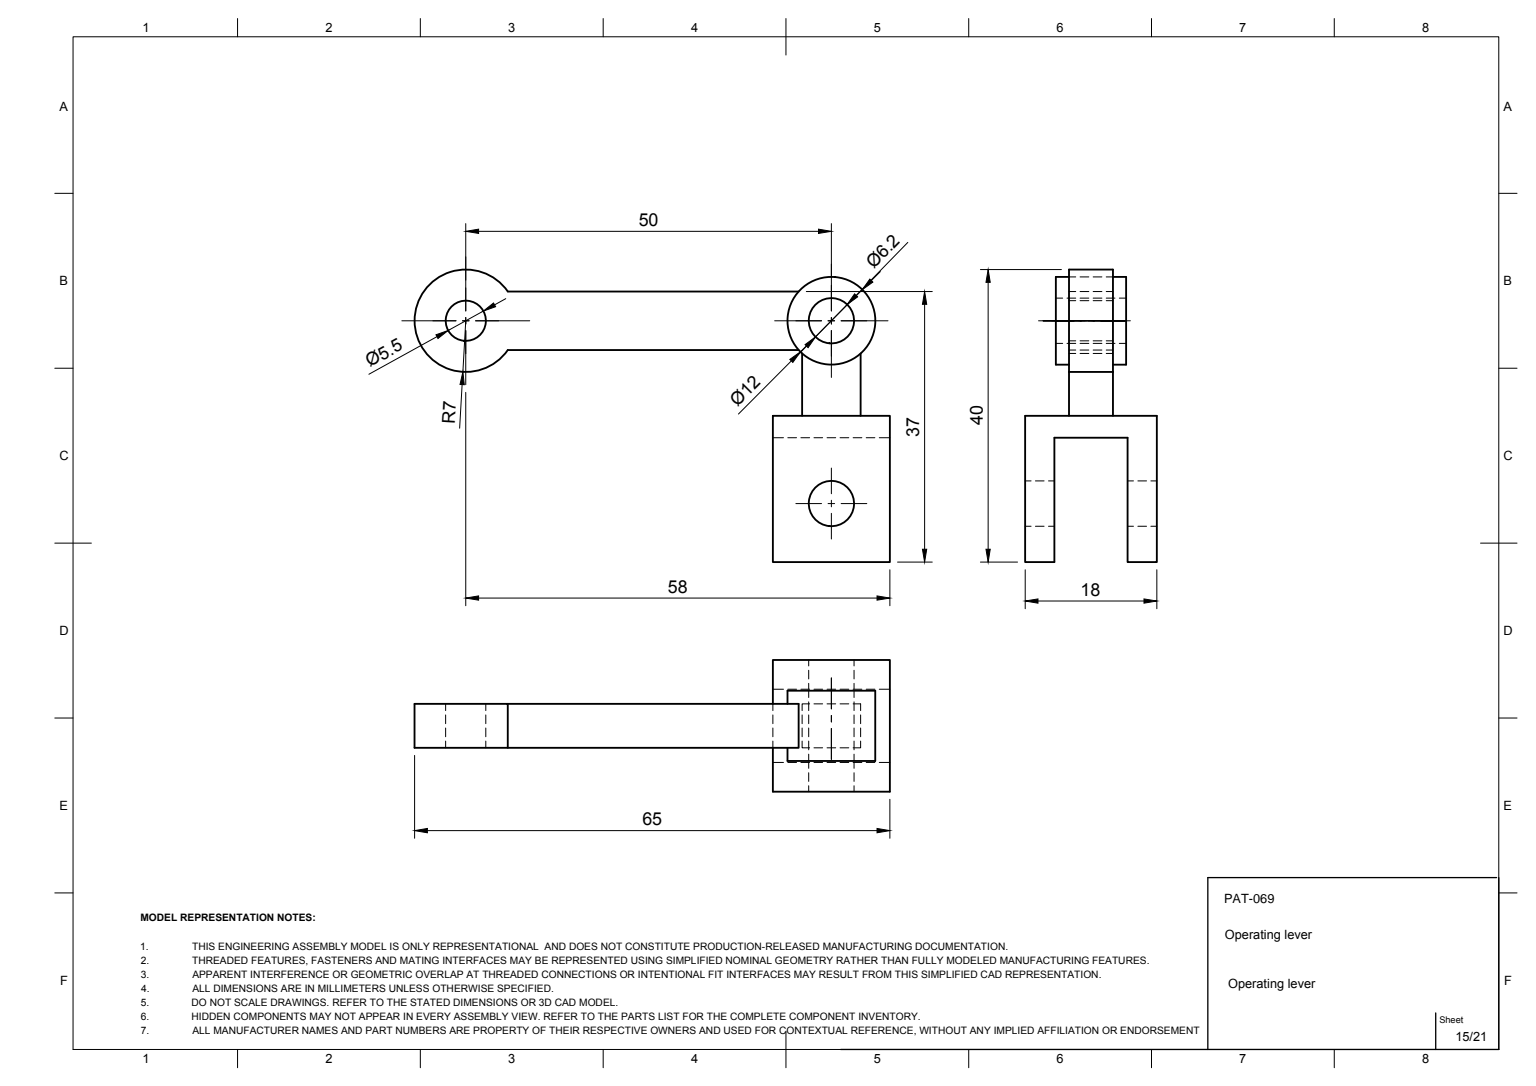
ISO-10303-21;
HEADER;
/* Generated by software containing ST-Developer
 * from STEP Tools, Inc. (www.steptools.com) 
 */

FILE_DESCRIPTION(
/* description */ ('Located fixture plate with toggle clamp'),
/* implementation_level */ '2;1');

FILE_NAME(
/* name */ 'Operating lever.step',
/* time_stamp */ '2026-10-27T21:36:12-07:00',
/* author */ (''),
/* organization */ (''),
/* preprocessor_version */ 'ST-DEVELOPER v20.2',
/* originating_system */ 'Autodesk Translation Framework v15.17.0.0',
/* authorisation */ '');

FILE_SCHEMA (('AUTOMOTIVE_DESIGN { 1 0 10303 214 3 1 1 }'));
ENDSEC;

DATA;
#10=MECHANICAL_DESIGN_GEOMETRIC_PRESENTATION_REPRESENTATION('',(#333),#9285);
#285=SHAPE_REPRESENTATION_RELATIONSHIP('SRR','None',#9409,#309);
#309=ADVANCED_BREP_SHAPE_REPRESENTATION('',(#355),#9271);
#333=STYLED_ITEM('',(#9598),#355);
#355=MANIFOLD_SOLID_BREP('Body1',#5183);
#453=FACE_BOUND('',#1236,.T.);
#454=FACE_BOUND('',#1239,.T.);
#455=FACE_BOUND('',#1245,.T.);
#456=FACE_BOUND('',#1248,.T.);
#457=FACE_BOUND('',#1254,.T.);
#458=FACE_BOUND('',#1255,.T.);
#459=FACE_BOUND('',#1257,.T.);
#460=FACE_BOUND('',#1259,.T.);
#461=FACE_BOUND('',#1262,.T.);
#462=FACE_BOUND('',#1264,.T.);
#463=FACE_BOUND('',#1268,.T.);
#594=PLANE('',#5789);
#595=PLANE('',#5791);
#596=PLANE('',#5792);
#597=PLANE('',#5794);
#598=PLANE('',#5801);
#599=PLANE('',#5802);
#600=PLANE('',#5803);
#601=PLANE('',#5804);
#602=PLANE('',#5805);
#603=PLANE('',#5807);
#604=PLANE('',#5808);
#605=PLANE('',#5810);
#606=PLANE('',#5814);
#607=PLANE('',#5815);
#608=PLANE('',#5816);
#609=PLANE('',#5817);
#610=PLANE('',#5818);
#611=PLANE('',#5819);
#612=PLANE('',#5820);
#613=PLANE('',#5821);
#850=FACE_OUTER_BOUND('',#1232,.T.);
#851=FACE_OUTER_BOUND('',#1233,.T.);
#852=FACE_OUTER_BOUND('',#1234,.T.);
#853=FACE_OUTER_BOUND('',#1235,.T.);
#854=FACE_OUTER_BOUND('',#1237,.T.);
#855=FACE_OUTER_BOUND('',#1238,.T.);
#856=FACE_OUTER_BOUND('',#1240,.T.);
#857=FACE_OUTER_BOUND('',#1241,.T.);
#858=FACE_OUTER_BOUND('',#1242,.T.);
#859=FACE_OUTER_BOUND('',#1243,.T.);
#860=FACE_OUTER_BOUND('',#1244,.T.);
#861=FACE_OUTER_BOUND('',#1246,.T.);
#862=FACE_OUTER_BOUND('',#1247,.T.);
#863=FACE_OUTER_BOUND('',#1249,.T.);
#864=FACE_OUTER_BOUND('',#1250,.T.);
#865=FACE_OUTER_BOUND('',#1251,.T.);
#866=FACE_OUTER_BOUND('',#1252,.T.);
#867=FACE_OUTER_BOUND('',#1253,.T.);
#868=FACE_OUTER_BOUND('',#1256,.T.);
#869=FACE_OUTER_BOUND('',#1258,.T.);
#870=FACE_OUTER_BOUND('',#1260,.T.);
#871=FACE_OUTER_BOUND('',#1261,.T.);
#872=FACE_OUTER_BOUND('',#1263,.T.);
#873=FACE_OUTER_BOUND('',#1265,.T.);
#874=FACE_OUTER_BOUND('',#1266,.T.);
#875=FACE_OUTER_BOUND('',#1267,.T.);
#1232=EDGE_LOOP('',(#4300,#4301,#4302,#4303));
#1233=EDGE_LOOP('',(#4304,#4305,#4306,#4307));
#1234=EDGE_LOOP('',(#4308,#4309,#4310,#4311));
#1235=EDGE_LOOP('',(#4312,#4313,#4314,#4315));
#1236=EDGE_LOOP('',(#4316));
#1237=EDGE_LOOP('',(#4317,#4318,#4319,#4320));
#1238=EDGE_LOOP('',(#4321,#4322,#4323,#4324));
#1239=EDGE_LOOP('',(#4325));
#1240=EDGE_LOOP('',(#4326,#4327,#4328,#4329));
#1241=EDGE_LOOP('',(#4330,#4331,#4332,#4333));
#1242=EDGE_LOOP('',(#4334,#4335,#4336,#4337));
#1243=EDGE_LOOP('',(#4338,#4339,#4340,#4341));
#1244=EDGE_LOOP('',(#4342,#4343,#4344,#4345));
#1245=EDGE_LOOP('',(#4346));
#1246=EDGE_LOOP('',(#4347,#4348,#4349,#4350));
#1247=EDGE_LOOP('',(#4351,#4352,#4353,#4354));
#1248=EDGE_LOOP('',(#4355));
#1249=EDGE_LOOP('',(#4356,#4357,#4358,#4359));
#1250=EDGE_LOOP('',(#4360,#4361,#4362,#4363));
#1251=EDGE_LOOP('',(#4364,#4365,#4366,#4367));
#1252=EDGE_LOOP('',(#4368,#4369,#4370,#4371));
#1253=EDGE_LOOP('',(#4372,#4373,#4374,#4375));
#1254=EDGE_LOOP('',(#4376,#4377,#4378,#4379));
#1255=EDGE_LOOP('',(#4380,#4381,#4382,#4383));
#1256=EDGE_LOOP('',(#4384));
#1257=EDGE_LOOP('',(#4385));
#1258=EDGE_LOOP('',(#4386));
#1259=EDGE_LOOP('',(#4387));
#1260=EDGE_LOOP('',(#4388,#4389,#4390,#4391,#4392,#4393,#4394,#4395));
#1261=EDGE_LOOP('',(#4396,#4397,#4398,#4399));
#1262=EDGE_LOOP('',(#4400));
#1263=EDGE_LOOP('',(#4401,#4402,#4403,#4404));
#1264=EDGE_LOOP('',(#4405,#4406,#4407,#4408));
#1265=EDGE_LOOP('',(#4409,#4410,#4411,#4412));
#1266=EDGE_LOOP('',(#4413,#4414,#4415,#4416,#4417,#4418,#4419,#4420));
#1267=EDGE_LOOP('',(#4421,#4422,#4423,#4424));
#1268=EDGE_LOOP('',(#4425));
#1509=CIRCLE('',#5781,0.275);
#1510=CIRCLE('',#5782,0.275);
#1511=CIRCLE('',#5784,0.31);
#1512=CIRCLE('',#5785,0.31);
#1513=CIRCLE('',#5787,0.7);
#1514=CIRCLE('',#5788,0.7);
#1515=CIRCLE('',#5790,0.6);
#1516=CIRCLE('',#5793,0.6);
#1517=CIRCLE('',#5796,0.31);
#1518=CIRCLE('',#5797,0.31);
#1519=CIRCLE('',#5799,0.31);
#1520=CIRCLE('',#5800,0.31);
#1521=CIRCLE('',#5806,0.6);
#1522=CIRCLE('',#5809,0.6);
#1523=CIRCLE('',#5812,0.6);
#1524=CIRCLE('',#5813,0.6);
#1841=LINE('',#8492,#2251);
#1842=LINE('',#8498,#2252);
#1843=LINE('',#8503,#2253);
#1844=LINE('',#8507,#2254);
#1845=LINE('',#8511,#2255);
#1846=LINE('',#8514,#2256);
#1847=LINE('',#8517,#2257);
#1848=LINE('',#8518,#2258);
#1849=LINE('',#8521,#2259);
#1850=LINE('',#8524,#2260);
#1851=LINE('',#8529,#2261);
#1852=LINE('',#8535,#2262);
#1853=LINE('',#8540,#2263);
#1854=LINE('',#8542,#2264);
#1855=LINE('',#8544,#2265);
#1856=LINE('',#8545,#2266);
#1857=LINE('',#8549,#2267);
#1858=LINE('',#8551,#2268);
#1859=LINE('',#8553,#2269);
#1860=LINE('',#8554,#2270);
#1861=LINE('',#8558,#2271);
#1862=LINE('',#8559,#2272);
#1863=LINE('',#8560,#2273);
#1864=LINE('',#8562,#2274);
#1865=LINE('',#8563,#2275);
#1866=LINE('',#8567,#2276);
#1867=LINE('',#8569,#2277);
#1868=LINE('',#8572,#2278);
#1869=LINE('',#8575,#2279);
#1870=LINE('',#8577,#2280);
#1871=LINE('',#8578,#2281);
#1872=LINE('',#8581,#2282);
#1873=LINE('',#8583,#2283);
#1874=LINE('',#8586,#2284);
#1875=LINE('',#8587,#2285);
#1876=LINE('',#8592,#2286);
#1877=LINE('',#8598,#2287);
#1878=LINE('',#8600,#2288);
#1879=LINE('',#8602,#2289);
#1880=LINE('',#8603,#2290);
#1881=LINE('',#8606,#2291);
#1882=LINE('',#8607,#2292);
#1883=LINE('',#8610,#2293);
#1884=LINE('',#8611,#2294);
#1885=LINE('',#8614,#2295);
#1886=LINE('',#8615,#2296);
#1887=LINE('',#8617,#2297);
#2251=VECTOR('',#6931,0.275);
#2252=VECTOR('',#6938,0.31);
#2253=VECTOR('',#6943,1.);
#2254=VECTOR('',#6946,1.);
#2255=VECTOR('',#6951,1.);
#2256=VECTOR('',#6954,1.);
#2257=VECTOR('',#6957,1.);
#2258=VECTOR('',#6958,1.);
#2259=VECTOR('',#6961,1.);
#2260=VECTOR('',#6966,1.);
#2261=VECTOR('',#6971,0.31);
#2262=VECTOR('',#6978,0.31);
#2263=VECTOR('',#6983,1.);
#2264=VECTOR('',#6984,1.);
#2265=VECTOR('',#6985,1.);
#2266=VECTOR('',#6986,1.);
#2267=VECTOR('',#6989,1.);
#2268=VECTOR('',#6990,1.);
#2269=VECTOR('',#6991,1.);
#2270=VECTOR('',#6992,1.);
#2271=VECTOR('',#6995,1.);
#2272=VECTOR('',#6996,1.);
#2273=VECTOR('',#6997,1.);
#2274=VECTOR('',#7000,1.);
#2275=VECTOR('',#7001,1.);
#2276=VECTOR('',#7004,1.);
#2277=VECTOR('',#7005,1.);
#2278=VECTOR('',#7008,1.);
#2279=VECTOR('',#7011,1.);
#2280=VECTOR('',#7012,1.);
#2281=VECTOR('',#7013,1.);
#2282=VECTOR('',#7016,1.);
#2283=VECTOR('',#7017,1.);
#2284=VECTOR('',#7022,1.);
#2285=VECTOR('',#7023,1.);
#2286=VECTOR('',#7028,0.6);
#2287=VECTOR('',#7037,1.);
#2288=VECTOR('',#7038,1.);
#2289=VECTOR('',#7039,1.);
#2290=VECTOR('',#7040,1.);
#2291=VECTOR('',#7043,1.);
#2292=VECTOR('',#7044,1.);
#2293=VECTOR('',#7047,1.);
#2294=VECTOR('',#7048,1.);
#2295=VECTOR('',#7051,1.);
#2296=VECTOR('',#7052,1.);
#2297=VECTOR('',#7055,1.);
#2669=VERTEX_POINT('',#8489);
#2670=VERTEX_POINT('',#8491);
#2671=VERTEX_POINT('',#8495);
#2672=VERTEX_POINT('',#8497);
#2673=VERTEX_POINT('',#8501);
#2674=VERTEX_POINT('',#8502);
#2675=VERTEX_POINT('',#8504);
#2676=VERTEX_POINT('',#8506);
#2677=VERTEX_POINT('',#8510);
#2678=VERTEX_POINT('',#8512);
#2679=VERTEX_POINT('',#8516);
#2680=VERTEX_POINT('',#8520);
#2681=VERTEX_POINT('',#8526);
#2682=VERTEX_POINT('',#8528);
#2683=VERTEX_POINT('',#8532);
#2684=VERTEX_POINT('',#8534);
#2685=VERTEX_POINT('',#8538);
#2686=VERTEX_POINT('',#8539);
#2687=VERTEX_POINT('',#8541);
#2688=VERTEX_POINT('',#8543);
#2689=VERTEX_POINT('',#8547);
#2690=VERTEX_POINT('',#8548);
#2691=VERTEX_POINT('',#8550);
#2692=VERTEX_POINT('',#8552);
#2693=VERTEX_POINT('',#8556);
#2694=VERTEX_POINT('',#8557);
#2695=VERTEX_POINT('',#8565);
#2696=VERTEX_POINT('',#8566);
#2697=VERTEX_POINT('',#8568);
#2698=VERTEX_POINT('',#8570);
#2699=VERTEX_POINT('',#8574);
#2700=VERTEX_POINT('',#8576);
#2701=VERTEX_POINT('',#8580);
#2702=VERTEX_POINT('',#8582);
#2703=VERTEX_POINT('',#8589);
#2704=VERTEX_POINT('',#8591);
#2705=VERTEX_POINT('',#8597);
#2706=VERTEX_POINT('',#8599);
#2707=VERTEX_POINT('',#8601);
#2708=VERTEX_POINT('',#8605);
#2709=VERTEX_POINT('',#8609);
#2710=VERTEX_POINT('',#8613);
#3238=EDGE_CURVE('',#2669,#2669,#1509,.T.);
#3239=EDGE_CURVE('',#2669,#2670,#1841,.T.);
#3240=EDGE_CURVE('',#2670,#2670,#1510,.T.);
#3241=EDGE_CURVE('',#2671,#2671,#1511,.T.);
#3242=EDGE_CURVE('',#2671,#2672,#1842,.T.);
#3243=EDGE_CURVE('',#2672,#2672,#1512,.T.);
#3244=EDGE_CURVE('',#2673,#2674,#1843,.T.);
#3245=EDGE_CURVE('',#2675,#2673,#1513,.T.);
#3246=EDGE_CURVE('',#2676,#2675,#1844,.T.);
#3247=EDGE_CURVE('',#2676,#2674,#1514,.T.);
#3248=EDGE_CURVE('',#2677,#2676,#1845,.T.);
#3249=EDGE_CURVE('',#2678,#2677,#1515,.T.);
#3250=EDGE_CURVE('',#2674,#2678,#1846,.T.);
#3251=EDGE_CURVE('',#2679,#2675,#1847,.T.);
#3252=EDGE_CURVE('',#2677,#2679,#1848,.T.);
#3253=EDGE_CURVE('',#2673,#2680,#1849,.T.);
#3254=EDGE_CURVE('',#2679,#2680,#1516,.T.);
#3255=EDGE_CURVE('',#2680,#2678,#1850,.T.);
#3256=EDGE_CURVE('',#2681,#2681,#1517,.T.);
#3257=EDGE_CURVE('',#2681,#2682,#1851,.T.);
#3258=EDGE_CURVE('',#2682,#2682,#1518,.T.);
#3259=EDGE_CURVE('',#2683,#2683,#1519,.T.);
#3260=EDGE_CURVE('',#2683,#2684,#1852,.T.);
#3261=EDGE_CURVE('',#2684,#2684,#1520,.T.);
#3262=EDGE_CURVE('',#2685,#2686,#1853,.T.);
#3263=EDGE_CURVE('',#2685,#2687,#1854,.T.);
#3264=EDGE_CURVE('',#2688,#2687,#1855,.T.);
#3265=EDGE_CURVE('',#2686,#2688,#1856,.T.);
#3266=EDGE_CURVE('',#2689,#2690,#1857,.T.);
#3267=EDGE_CURVE('',#2690,#2691,#1858,.T.);
#3268=EDGE_CURVE('',#2691,#2692,#1859,.T.);
#3269=EDGE_CURVE('',#2692,#2689,#1860,.T.);
#3270=EDGE_CURVE('',#2693,#2694,#1861,.T.);
#3271=EDGE_CURVE('',#2693,#2691,#1862,.T.);
#3272=EDGE_CURVE('',#2694,#2690,#1863,.T.);
#3273=EDGE_CURVE('',#2687,#2693,#1864,.T.);
#3274=EDGE_CURVE('',#2694,#2688,#1865,.T.);
#3275=EDGE_CURVE('',#2695,#2696,#1866,.T.);
#3276=EDGE_CURVE('',#2697,#2696,#1867,.T.);
#3277=EDGE_CURVE('',#2698,#2697,#1521,.T.);
#3278=EDGE_CURVE('',#2695,#2698,#1868,.T.);
#3279=EDGE_CURVE('',#2696,#2699,#1869,.T.);
#3280=EDGE_CURVE('',#2700,#2699,#1870,.T.);
#3281=EDGE_CURVE('',#2697,#2700,#1871,.T.);
#3282=EDGE_CURVE('',#2699,#2701,#1872,.T.);
#3283=EDGE_CURVE('',#2701,#2702,#1873,.T.);
#3284=EDGE_CURVE('',#2700,#2702,#1522,.T.);
#3285=EDGE_CURVE('',#2701,#2695,#1874,.T.);
#3286=EDGE_CURVE('',#2702,#2698,#1875,.T.);
#3287=EDGE_CURVE('',#2703,#2703,#1523,.T.);
#3288=EDGE_CURVE('',#2703,#2704,#1876,.T.);
#3289=EDGE_CURVE('',#2704,#2704,#1524,.T.);
#3290=EDGE_CURVE('',#2705,#2685,#1877,.T.);
#3291=EDGE_CURVE('',#2706,#2705,#1878,.T.);
#3292=EDGE_CURVE('',#2707,#2706,#1879,.T.);
#3293=EDGE_CURVE('',#2707,#2692,#1880,.T.);
#3294=EDGE_CURVE('',#2686,#2708,#1881,.T.);
#3295=EDGE_CURVE('',#2708,#2705,#1882,.T.);
#3296=EDGE_CURVE('',#2709,#2707,#1883,.T.);
#3297=EDGE_CURVE('',#2709,#2689,#1884,.T.);
#3298=EDGE_CURVE('',#2706,#2710,#1885,.T.);
#3299=EDGE_CURVE('',#2710,#2708,#1886,.T.);
#3300=EDGE_CURVE('',#2710,#2709,#1887,.T.);
#4300=ORIENTED_EDGE('',*,*,#3238,.F.);
#4301=ORIENTED_EDGE('',*,*,#3239,.T.);
#4302=ORIENTED_EDGE('',*,*,#3240,.F.);
#4303=ORIENTED_EDGE('',*,*,#3239,.F.);
#4304=ORIENTED_EDGE('',*,*,#3241,.F.);
#4305=ORIENTED_EDGE('',*,*,#3242,.T.);
#4306=ORIENTED_EDGE('',*,*,#3243,.F.);
#4307=ORIENTED_EDGE('',*,*,#3242,.F.);
#4308=ORIENTED_EDGE('',*,*,#3244,.F.);
#4309=ORIENTED_EDGE('',*,*,#3245,.F.);
#4310=ORIENTED_EDGE('',*,*,#3246,.F.);
#4311=ORIENTED_EDGE('',*,*,#3247,.T.);
#4312=ORIENTED_EDGE('',*,*,#3247,.F.);
#4313=ORIENTED_EDGE('',*,*,#3248,.F.);
#4314=ORIENTED_EDGE('',*,*,#3249,.F.);
#4315=ORIENTED_EDGE('',*,*,#3250,.F.);
#4316=ORIENTED_EDGE('',*,*,#3238,.T.);
#4317=ORIENTED_EDGE('',*,*,#3246,.T.);
#4318=ORIENTED_EDGE('',*,*,#3251,.F.);
#4319=ORIENTED_EDGE('',*,*,#3252,.F.);
#4320=ORIENTED_EDGE('',*,*,#3248,.T.);
#4321=ORIENTED_EDGE('',*,*,#3253,.T.);
#4322=ORIENTED_EDGE('',*,*,#3254,.F.);
#4323=ORIENTED_EDGE('',*,*,#3251,.T.);
#4324=ORIENTED_EDGE('',*,*,#3245,.T.);
#4325=ORIENTED_EDGE('',*,*,#3240,.T.);
#4326=ORIENTED_EDGE('',*,*,#3244,.T.);
#4327=ORIENTED_EDGE('',*,*,#3250,.T.);
#4328=ORIENTED_EDGE('',*,*,#3255,.F.);
#4329=ORIENTED_EDGE('',*,*,#3253,.F.);
#4330=ORIENTED_EDGE('',*,*,#3256,.F.);
#4331=ORIENTED_EDGE('',*,*,#3257,.T.);
#4332=ORIENTED_EDGE('',*,*,#3258,.F.);
#4333=ORIENTED_EDGE('',*,*,#3257,.F.);
#4334=ORIENTED_EDGE('',*,*,#3259,.F.);
#4335=ORIENTED_EDGE('',*,*,#3260,.T.);
#4336=ORIENTED_EDGE('',*,*,#3261,.F.);
#4337=ORIENTED_EDGE('',*,*,#3260,.F.);
#4338=ORIENTED_EDGE('',*,*,#3262,.F.);
#4339=ORIENTED_EDGE('',*,*,#3263,.T.);
#4340=ORIENTED_EDGE('',*,*,#3264,.F.);
#4341=ORIENTED_EDGE('',*,*,#3265,.F.);
#4342=ORIENTED_EDGE('',*,*,#3266,.T.);
#4343=ORIENTED_EDGE('',*,*,#3267,.T.);
#4344=ORIENTED_EDGE('',*,*,#3268,.T.);
#4345=ORIENTED_EDGE('',*,*,#3269,.T.);
#4346=ORIENTED_EDGE('',*,*,#3261,.T.);
#4347=ORIENTED_EDGE('',*,*,#3270,.F.);
#4348=ORIENTED_EDGE('',*,*,#3271,.T.);
#4349=ORIENTED_EDGE('',*,*,#3267,.F.);
#4350=ORIENTED_EDGE('',*,*,#3272,.F.);
#4351=ORIENTED_EDGE('',*,*,#3264,.T.);
#4352=ORIENTED_EDGE('',*,*,#3273,.T.);
#4353=ORIENTED_EDGE('',*,*,#3270,.T.);
#4354=ORIENTED_EDGE('',*,*,#3274,.T.);
#4355=ORIENTED_EDGE('',*,*,#3259,.T.);
#4356=ORIENTED_EDGE('',*,*,#3275,.T.);
#4357=ORIENTED_EDGE('',*,*,#3276,.F.);
#4358=ORIENTED_EDGE('',*,*,#3277,.F.);
#4359=ORIENTED_EDGE('',*,*,#3278,.F.);
#4360=ORIENTED_EDGE('',*,*,#3279,.T.);
#4361=ORIENTED_EDGE('',*,*,#3280,.F.);
#4362=ORIENTED_EDGE('',*,*,#3281,.F.);
#4363=ORIENTED_EDGE('',*,*,#3276,.T.);
#4364=ORIENTED_EDGE('',*,*,#3282,.T.);
#4365=ORIENTED_EDGE('',*,*,#3283,.T.);
#4366=ORIENTED_EDGE('',*,*,#3284,.F.);
#4367=ORIENTED_EDGE('',*,*,#3280,.T.);
#4368=ORIENTED_EDGE('',*,*,#3285,.T.);
#4369=ORIENTED_EDGE('',*,*,#3278,.T.);
#4370=ORIENTED_EDGE('',*,*,#3286,.F.);
#4371=ORIENTED_EDGE('',*,*,#3283,.F.);
#4372=ORIENTED_EDGE('',*,*,#3287,.F.);
#4373=ORIENTED_EDGE('',*,*,#3288,.T.);
#4374=ORIENTED_EDGE('',*,*,#3289,.T.);
#4375=ORIENTED_EDGE('',*,*,#3288,.F.);
#4376=ORIENTED_EDGE('',*,*,#3252,.T.);
#4377=ORIENTED_EDGE('',*,*,#3254,.T.);
#4378=ORIENTED_EDGE('',*,*,#3255,.T.);
#4379=ORIENTED_EDGE('',*,*,#3249,.T.);
#4380=ORIENTED_EDGE('',*,*,#3281,.T.);
#4381=ORIENTED_EDGE('',*,*,#3284,.T.);
#4382=ORIENTED_EDGE('',*,*,#3286,.T.);
#4383=ORIENTED_EDGE('',*,*,#3277,.T.);
#4384=ORIENTED_EDGE('',*,*,#3287,.T.);
#4385=ORIENTED_EDGE('',*,*,#3243,.T.);
#4386=ORIENTED_EDGE('',*,*,#3289,.F.);
#4387=ORIENTED_EDGE('',*,*,#3241,.T.);
#4388=ORIENTED_EDGE('',*,*,#3290,.F.);
#4389=ORIENTED_EDGE('',*,*,#3291,.F.);
#4390=ORIENTED_EDGE('',*,*,#3292,.F.);
#4391=ORIENTED_EDGE('',*,*,#3293,.T.);
#4392=ORIENTED_EDGE('',*,*,#3268,.F.);
#4393=ORIENTED_EDGE('',*,*,#3271,.F.);
#4394=ORIENTED_EDGE('',*,*,#3273,.F.);
#4395=ORIENTED_EDGE('',*,*,#3263,.F.);
#4396=ORIENTED_EDGE('',*,*,#3262,.T.);
#4397=ORIENTED_EDGE('',*,*,#3294,.T.);
#4398=ORIENTED_EDGE('',*,*,#3295,.T.);
#4399=ORIENTED_EDGE('',*,*,#3290,.T.);
#4400=ORIENTED_EDGE('',*,*,#3258,.T.);
#4401=ORIENTED_EDGE('',*,*,#3296,.F.);
#4402=ORIENTED_EDGE('',*,*,#3297,.T.);
#4403=ORIENTED_EDGE('',*,*,#3269,.F.);
#4404=ORIENTED_EDGE('',*,*,#3293,.F.);
#4405=ORIENTED_EDGE('',*,*,#3282,.F.);
#4406=ORIENTED_EDGE('',*,*,#3279,.F.);
#4407=ORIENTED_EDGE('',*,*,#3275,.F.);
#4408=ORIENTED_EDGE('',*,*,#3285,.F.);
#4409=ORIENTED_EDGE('',*,*,#3298,.F.);
#4410=ORIENTED_EDGE('',*,*,#3291,.T.);
#4411=ORIENTED_EDGE('',*,*,#3295,.F.);
#4412=ORIENTED_EDGE('',*,*,#3299,.F.);
#4413=ORIENTED_EDGE('',*,*,#3300,.F.);
#4414=ORIENTED_EDGE('',*,*,#3299,.T.);
#4415=ORIENTED_EDGE('',*,*,#3294,.F.);
#4416=ORIENTED_EDGE('',*,*,#3265,.T.);
#4417=ORIENTED_EDGE('',*,*,#3274,.F.);
#4418=ORIENTED_EDGE('',*,*,#3272,.T.);
#4419=ORIENTED_EDGE('',*,*,#3266,.F.);
#4420=ORIENTED_EDGE('',*,*,#3297,.F.);
#4421=ORIENTED_EDGE('',*,*,#3292,.T.);
#4422=ORIENTED_EDGE('',*,*,#3298,.T.);
#4423=ORIENTED_EDGE('',*,*,#3300,.T.);
#4424=ORIENTED_EDGE('',*,*,#3296,.T.);
#4425=ORIENTED_EDGE('',*,*,#3256,.T.);
#4845=CYLINDRICAL_SURFACE('',#5780,0.275);
#4846=CYLINDRICAL_SURFACE('',#5783,0.31);
#4847=CYLINDRICAL_SURFACE('',#5786,0.7);
#4848=CYLINDRICAL_SURFACE('',#5795,0.31);
#4849=CYLINDRICAL_SURFACE('',#5798,0.31);
#4850=CYLINDRICAL_SURFACE('',#5811,0.6);
#5051=ADVANCED_FACE('',(#850),#4845,.F.);
#5052=ADVANCED_FACE('',(#851),#4846,.F.);
#5053=ADVANCED_FACE('',(#852),#4847,.T.);
#5054=ADVANCED_FACE('',(#853,#453),#594,.F.);
#5055=ADVANCED_FACE('',(#854),#595,.T.);
#5056=ADVANCED_FACE('',(#855,#454),#596,.T.);
#5057=ADVANCED_FACE('',(#856),#597,.T.);
#5058=ADVANCED_FACE('',(#857),#4848,.F.);
#5059=ADVANCED_FACE('',(#858),#4849,.F.);
#5060=ADVANCED_FACE('',(#859),#598,.T.);
#5061=ADVANCED_FACE('',(#860,#455),#599,.T.);
#5062=ADVANCED_FACE('',(#861),#600,.T.);
#5063=ADVANCED_FACE('',(#862,#456),#601,.F.);
#5064=ADVANCED_FACE('',(#863),#602,.F.);
#5065=ADVANCED_FACE('',(#864),#603,.T.);
#5066=ADVANCED_FACE('',(#865),#604,.T.);
#5067=ADVANCED_FACE('',(#866),#605,.T.);
#5068=ADVANCED_FACE('',(#867,#457,#458),#4850,.T.);
#5069=ADVANCED_FACE('',(#868,#459),#606,.T.);
#5070=ADVANCED_FACE('',(#869,#460),#607,.F.);
#5071=ADVANCED_FACE('',(#870),#608,.T.);
#5072=ADVANCED_FACE('',(#871,#461),#609,.T.);
#5073=ADVANCED_FACE('',(#872,#462),#610,.T.);
#5074=ADVANCED_FACE('',(#873),#611,.T.);
#5075=ADVANCED_FACE('',(#874),#612,.T.);
#5076=ADVANCED_FACE('',(#875,#463),#613,.F.);
#5183=CLOSED_SHELL('',(#5051,#5052,#5053,#5054,#5055,#5056,#5057,#5058,
#5059,#5060,#5061,#5062,#5063,#5064,#5065,#5066,#5067,#5068,#5069,#5070,
#5071,#5072,#5073,#5074,#5075,#5076));
#5779=AXIS2_PLACEMENT_3D('',#8487,#6925,#6926);
#5780=AXIS2_PLACEMENT_3D('',#8488,#6927,#6928);
#5781=AXIS2_PLACEMENT_3D('',#8490,#6929,#6930);
#5782=AXIS2_PLACEMENT_3D('',#8493,#6932,#6933);
#5783=AXIS2_PLACEMENT_3D('',#8494,#6934,#6935);
#5784=AXIS2_PLACEMENT_3D('',#8496,#6936,#6937);
#5785=AXIS2_PLACEMENT_3D('',#8499,#6939,#6940);
#5786=AXIS2_PLACEMENT_3D('',#8500,#6941,#6942);
#5787=AXIS2_PLACEMENT_3D('',#8505,#6944,#6945);
#5788=AXIS2_PLACEMENT_3D('',#8508,#6947,#6948);
#5789=AXIS2_PLACEMENT_3D('',#8509,#6949,#6950);
#5790=AXIS2_PLACEMENT_3D('',#8513,#6952,#6953);
#5791=AXIS2_PLACEMENT_3D('',#8515,#6955,#6956);
#5792=AXIS2_PLACEMENT_3D('',#8519,#6959,#6960);
#5793=AXIS2_PLACEMENT_3D('',#8522,#6962,#6963);
#5794=AXIS2_PLACEMENT_3D('',#8523,#6964,#6965);
#5795=AXIS2_PLACEMENT_3D('',#8525,#6967,#6968);
#5796=AXIS2_PLACEMENT_3D('',#8527,#6969,#6970);
#5797=AXIS2_PLACEMENT_3D('',#8530,#6972,#6973);
#5798=AXIS2_PLACEMENT_3D('',#8531,#6974,#6975);
#5799=AXIS2_PLACEMENT_3D('',#8533,#6976,#6977);
#5800=AXIS2_PLACEMENT_3D('',#8536,#6979,#6980);
#5801=AXIS2_PLACEMENT_3D('',#8537,#6981,#6982);
#5802=AXIS2_PLACEMENT_3D('',#8546,#6987,#6988);
#5803=AXIS2_PLACEMENT_3D('',#8555,#6993,#6994);
#5804=AXIS2_PLACEMENT_3D('',#8561,#6998,#6999);
#5805=AXIS2_PLACEMENT_3D('',#8564,#7002,#7003);
#5806=AXIS2_PLACEMENT_3D('',#8571,#7006,#7007);
#5807=AXIS2_PLACEMENT_3D('',#8573,#7009,#7010);
#5808=AXIS2_PLACEMENT_3D('',#8579,#7014,#7015);
#5809=AXIS2_PLACEMENT_3D('',#8584,#7018,#7019);
#5810=AXIS2_PLACEMENT_3D('',#8585,#7020,#7021);
#5811=AXIS2_PLACEMENT_3D('',#8588,#7024,#7025);
#5812=AXIS2_PLACEMENT_3D('',#8590,#7026,#7027);
#5813=AXIS2_PLACEMENT_3D('',#8593,#7029,#7030);
#5814=AXIS2_PLACEMENT_3D('',#8594,#7031,#7032);
#5815=AXIS2_PLACEMENT_3D('',#8595,#7033,#7034);
#5816=AXIS2_PLACEMENT_3D('',#8596,#7035,#7036);
#5817=AXIS2_PLACEMENT_3D('',#8604,#7041,#7042);
#5818=AXIS2_PLACEMENT_3D('',#8608,#7045,#7046);
#5819=AXIS2_PLACEMENT_3D('',#8612,#7049,#7050);
#5820=AXIS2_PLACEMENT_3D('',#8616,#7053,#7054);
#5821=AXIS2_PLACEMENT_3D('',#8618,#7056,#7057);
#6925=DIRECTION('axis',(0.,0.,1.));
#6926=DIRECTION('refdir',(1.,0.,0.));
#6927=DIRECTION('center_axis',(0.,1.,0.));
#6928=DIRECTION('ref_axis',(1.,0.,0.));
#6929=DIRECTION('center_axis',(0.,1.,0.));
#6930=DIRECTION('ref_axis',(1.,0.,0.));
#6931=DIRECTION('',(0.,1.,0.));
#6932=DIRECTION('center_axis',(0.,-1.,0.));
#6933=DIRECTION('ref_axis',(1.,0.,0.));
#6934=DIRECTION('center_axis',(0.,1.,0.));
#6935=DIRECTION('ref_axis',(1.,0.,0.));
#6936=DIRECTION('center_axis',(0.,1.,0.));
#6937=DIRECTION('ref_axis',(1.,0.,0.));
#6938=DIRECTION('',(0.,1.,0.));
#6939=DIRECTION('center_axis',(0.,-1.,0.));
#6940=DIRECTION('ref_axis',(1.,0.,0.));
#6941=DIRECTION('center_axis',(0.,1.,0.));
#6942=DIRECTION('ref_axis',(0.0871557427476581,0.,0.996194698091746));
#6943=DIRECTION('',(0.,-1.,0.));
#6944=DIRECTION('center_axis',(0.,1.,0.));
#6945=DIRECTION('ref_axis',(1.,0.,0.));
#6946=DIRECTION('',(0.,1.,0.));
#6947=DIRECTION('center_axis',(0.,1.,0.));
#6948=DIRECTION('ref_axis',(1.,0.,0.));
#6949=DIRECTION('center_axis',(0.,1.,0.));
#6950=DIRECTION('ref_axis',(1.,0.,0.));
#6951=DIRECTION('',(0.0871557427476582,0.,0.996194698091746));
#6952=DIRECTION('center_axis',(0.,-1.,0.));
#6953=DIRECTION('ref_axis',(1.,0.,0.));
#6954=DIRECTION('',(-0.0871557427476581,0.,-0.996194698091746));
#6955=DIRECTION('center_axis',(-0.996194698091746,0.,0.0871557427476582));
#6956=DIRECTION('ref_axis',(0.0871557427476582,0.,0.996194698091746));
#6957=DIRECTION('',(0.0871557427476582,0.,0.996194698091746));
#6958=DIRECTION('',(0.,1.,0.));
#6959=DIRECTION('center_axis',(0.,1.,0.));
#6960=DIRECTION('ref_axis',(0.,0.,1.));
#6961=DIRECTION('',(-0.0871557427476581,0.,-0.996194698091746));
#6962=DIRECTION('center_axis',(0.,1.,0.));
#6963=DIRECTION('ref_axis',(1.,0.,0.));
#6964=DIRECTION('center_axis',(0.996194698091746,0.,-0.0871557427476581));
#6965=DIRECTION('ref_axis',(-0.0871557427476581,0.,-0.996194698091746));
#6966=DIRECTION('',(0.,-1.,0.));
#6967=DIRECTION('center_axis',(0.,1.,0.));
#6968=DIRECTION('ref_axis',(1.,0.,0.));
#6969=DIRECTION('center_axis',(0.,1.,0.));
#6970=DIRECTION('ref_axis',(1.,0.,0.));
#6971=DIRECTION('',(0.,1.,0.));
#6972=DIRECTION('center_axis',(0.,-1.,0.));
#6973=DIRECTION('ref_axis',(1.,0.,0.));
#6974=DIRECTION('center_axis',(0.,1.,0.));
#6975=DIRECTION('ref_axis',(1.,0.,0.));
#6976=DIRECTION('center_axis',(0.,1.,0.));
#6977=DIRECTION('ref_axis',(1.,0.,0.));
#6978=DIRECTION('',(0.,1.,0.));
#6979=DIRECTION('center_axis',(0.,-1.,0.));
#6980=DIRECTION('ref_axis',(1.,0.,0.));
#6981=DIRECTION('center_axis',(0.996194698091746,0.,-0.0871557427476583));
#6982=DIRECTION('ref_axis',(-0.0871557427476583,0.,-0.996194698091746));
#6983=DIRECTION('',(0.0871557427476583,0.,0.996194698091746));
#6984=DIRECTION('',(0.,1.,0.));
#6985=DIRECTION('',(-0.0871557427476583,0.,-0.996194698091746));
#6986=DIRECTION('',(0.,1.,0.));
#6987=DIRECTION('center_axis',(0.,1.,0.));
#6988=DIRECTION('ref_axis',(0.,0.,1.));
#6989=DIRECTION('',(0.996194698091746,0.,-0.0871557427476581));
#6990=DIRECTION('',(-0.087155742747658,0.,-0.996194698091746));
#6991=DIRECTION('',(-0.996194698091746,0.,0.0871557427476581));
#6992=DIRECTION('',(0.0871557427476582,0.,0.996194698091746));
#6993=DIRECTION('center_axis',(0.996194698091746,0.,-0.087155742747658));
#6994=DIRECTION('ref_axis',(-0.087155742747658,0.,-0.996194698091746));
#6995=DIRECTION('',(0.087155742747658,0.,0.996194698091746));
#6996=DIRECTION('',(0.,1.,0.));
#6997=DIRECTION('',(0.,1.,0.));
#6998=DIRECTION('center_axis',(0.,1.,0.));
#6999=DIRECTION('ref_axis',(1.,0.,0.));
#7000=DIRECTION('',(0.996194698091746,0.,-0.0871557427476581));
#7001=DIRECTION('',(-0.996194698091746,0.,0.0871557427476581));
#7002=DIRECTION('center_axis',(0.,1.,0.));
#7003=DIRECTION('ref_axis',(1.,0.,0.));
#7004=DIRECTION('',(0.0871557427476582,0.,0.996194698091746));
#7005=DIRECTION('',(0.996194698091746,0.,-0.0871557427476581));
#7006=DIRECTION('center_axis',(0.,-1.,0.));
#7007=DIRECTION('ref_axis',(1.,0.,0.));
#7008=DIRECTION('',(-0.996194698091746,0.,0.087155742747658));
#7009=DIRECTION('center_axis',(0.0871557427476581,0.,0.996194698091746));
#7010=DIRECTION('ref_axis',(0.996194698091746,0.,-0.0871557427476581));
#7011=DIRECTION('',(0.,1.,0.));
#7012=DIRECTION('',(0.996194698091746,0.,-0.0871557427476581));
#7013=DIRECTION('',(0.,1.,0.));
#7014=DIRECTION('center_axis',(0.,1.,0.));
#7015=DIRECTION('ref_axis',(0.,0.,1.));
#7016=DIRECTION('',(-0.0871557427476582,0.,-0.996194698091746));
#7017=DIRECTION('',(-0.996194698091746,0.,0.087155742747658));
#7018=DIRECTION('center_axis',(0.,1.,0.));
#7019=DIRECTION('ref_axis',(1.,0.,0.));
#7020=DIRECTION('center_axis',(-0.087155742747658,0.,-0.996194698091746));
#7021=DIRECTION('ref_axis',(-0.996194698091746,0.,0.087155742747658));
#7022=DIRECTION('',(0.,-1.,0.));
#7023=DIRECTION('',(0.,-1.,0.));
#7024=DIRECTION('center_axis',(0.,1.,0.));
#7025=DIRECTION('ref_axis',(1.,0.,0.));
#7026=DIRECTION('center_axis',(0.,1.,0.));
#7027=DIRECTION('ref_axis',(1.,0.,0.));
#7028=DIRECTION('',(0.,-1.,0.));
#7029=DIRECTION('center_axis',(0.,1.,0.));
#7030=DIRECTION('ref_axis',(1.,0.,0.));
#7031=DIRECTION('center_axis',(0.,1.,0.));
#7032=DIRECTION('ref_axis',(1.,0.,0.));
#7033=DIRECTION('center_axis',(0.,1.,0.));
#7034=DIRECTION('ref_axis',(1.,0.,0.));
#7035=DIRECTION('center_axis',(-0.0871557427476581,0.,-0.996194698091746));
#7036=DIRECTION('ref_axis',(-0.996194698091746,0.,0.0871557427476581));
#7037=DIRECTION('',(-0.996194698091746,0.,0.0871557427476581));
#7038=DIRECTION('',(0.,1.,0.));
#7039=DIRECTION('',(0.996194698091746,0.,-0.0871557427476581));
#7040=DIRECTION('',(0.,1.,0.));
#7041=DIRECTION('center_axis',(0.,1.,0.));
#7042=DIRECTION('ref_axis',(0.,0.,1.));
#7043=DIRECTION('',(0.996194698091746,0.,-0.0871557427476581));
#7044=DIRECTION('',(-0.087155742747658,0.,-0.996194698091746));
#7045=DIRECTION('center_axis',(-0.996194698091746,0.,0.0871557427476582));
#7046=DIRECTION('ref_axis',(0.0871557427476582,0.,0.996194698091746));
#7047=DIRECTION('',(-0.0871557427476582,0.,-0.996194698091746));
#7048=DIRECTION('',(0.,1.,0.));
#7049=DIRECTION('center_axis',(0.996194698091746,0.,-0.087155742747658));
#7050=DIRECTION('ref_axis',(-0.087155742747658,0.,-0.996194698091746));
#7051=DIRECTION('',(0.087155742747658,0.,0.996194698091746));
#7052=DIRECTION('',(0.,1.,0.));
#7053=DIRECTION('center_axis',(0.0871557427476581,0.,0.996194698091746));
#7054=DIRECTION('ref_axis',(0.996194698091746,0.,-0.0871557427476581));
#7055=DIRECTION('',(-0.996194698091746,0.,0.0871557427476581));
#7056=DIRECTION('center_axis',(0.,1.,0.));
#7057=DIRECTION('ref_axis',(1.,0.,0.));
#8487=CARTESIAN_POINT('',(0.,0.,0.));
#8488=CARTESIAN_POINT('Origin',(0.435778713738291,-0.4,7.48097349045873));
#8489=CARTESIAN_POINT('',(0.160778713738291,-0.3,7.48097349045873));
#8490=CARTESIAN_POINT('Origin',(0.435778713738291,-0.3,7.48097349045873));
#8491=CARTESIAN_POINT('',(0.160778713738291,0.3,7.48097349045873));
#8492=CARTESIAN_POINT('',(0.160778713738291,-0.4,7.48097349045873));
#8493=CARTESIAN_POINT('Origin',(0.435778713738291,0.3,7.48097349045873));
#8494=CARTESIAN_POINT('Origin',(0.,-0.6,2.5));
#8495=CARTESIAN_POINT('',(-0.31,-0.48,2.5));
#8496=CARTESIAN_POINT('Origin',(0.,-0.48,2.5));
#8497=CARTESIAN_POINT('',(-0.31,0.48,2.5));
#8498=CARTESIAN_POINT('',(-0.31,-0.6,2.5));
#8499=CARTESIAN_POINT('Origin',(0.,0.48,2.5));
#8500=CARTESIAN_POINT('Origin',(0.435778713738291,-0.3,7.48097349045873));
#8501=CARTESIAN_POINT('',(0.784189430553042,0.3,6.87384090822596));
#8502=CARTESIAN_POINT('',(0.784189430553042,-0.3,6.87384090822596));
#8503=CARTESIAN_POINT('',(0.784189430553042,-0.3,6.87384090822596));
#8504=CARTESIAN_POINT('',(-0.0127663279203548,0.3,6.94356550242408));
#8505=CARTESIAN_POINT('Origin',(0.435778713738291,0.3,7.48097349045873));
#8506=CARTESIAN_POINT('',(-0.0127663279203548,-0.3,6.94356550242408));
#8507=CARTESIAN_POINT('',(-0.0127663279203548,-0.3,6.94356550242408));
#8508=CARTESIAN_POINT('Origin',(0.435778713738291,-0.3,7.48097349045873));
#8509=CARTESIAN_POINT('Origin',(0.217889356869145,-0.3,4.99048674522937));
#8510=CARTESIAN_POINT('',(-0.359500646154049,-0.3,2.98037410985067));
#8511=CARTESIAN_POINT('',(-0.398477879236698,-0.3,2.53486229709906));
#8512=CARTESIAN_POINT('',(0.437455112319348,-0.3,2.91064951565254));
#8513=CARTESIAN_POINT('Origin',(0.,-0.3,2.5));
#8514=CARTESIAN_POINT('',(0.834256592974989,-0.3,7.44611119335967));
#8515=CARTESIAN_POINT('Origin',(-0.398477879236698,-0.3,2.53486229709906));
#8516=CARTESIAN_POINT('',(-0.359500646154049,0.3,2.98037410985067));
#8517=CARTESIAN_POINT('',(-0.398477879236698,0.3,2.53486229709906));
#8518=CARTESIAN_POINT('',(-0.359500646154049,-0.48,2.98037410985067));
#8519=CARTESIAN_POINT('Origin',(0.217889356869145,0.3,4.99048674522937));
#8520=CARTESIAN_POINT('',(0.437455112319348,0.3,2.91064951565254));
#8521=CARTESIAN_POINT('',(0.834256592974989,0.3,7.44611119335967));
#8522=CARTESIAN_POINT('Origin',(0.,0.3,2.5));
#8523=CARTESIAN_POINT('Origin',(0.834256592974989,-0.3,7.44611119335967));
#8524=CARTESIAN_POINT('',(0.437455112319348,-0.48,2.91064951565254));
#8525=CARTESIAN_POINT('Origin',(2.49048674522936,-1.,2.28211064313085));
#8526=CARTESIAN_POINT('',(2.18048674522936,-0.9,2.28211064313085));
#8527=CARTESIAN_POINT('Origin',(2.49048674522936,-0.9,2.28211064313085));
#8528=CARTESIAN_POINT('',(2.18048674522936,-0.5,2.28211064313085));
#8529=CARTESIAN_POINT('',(2.18048674522936,-1.,2.28211064313085));
#8530=CARTESIAN_POINT('Origin',(2.49048674522936,-0.5,2.28211064313085));
#8531=CARTESIAN_POINT('Origin',(2.49048674522936,-1.,2.28211064313085));
#8532=CARTESIAN_POINT('',(2.18048674522936,0.5,2.28211064313085));
#8533=CARTESIAN_POINT('Origin',(2.49048674522936,0.5,2.28211064313085));
#8534=CARTESIAN_POINT('',(2.18048674522936,0.9,2.28211064313085));
#8535=CARTESIAN_POINT('',(2.18048674522936,-1.,2.28211064313085));
#8536=CARTESIAN_POINT('Origin',(2.49048674522936,0.9,2.28211064313085));
#8537=CARTESIAN_POINT('Origin',(1.66363611114492,-0.9,3.15750657007714));
#8538=CARTESIAN_POINT('',(1.52418692274867,-0.5,1.56359505313035));
#8539=CARTESIAN_POINT('',(1.66363611114492,-0.5,3.15750657007714));
#8540=CARTESIAN_POINT('',(1.62877381404586,-0.5,2.75902869084045));
#8541=CARTESIAN_POINT('',(1.52418692274867,0.5,1.56359505313035));
#8542=CARTESIAN_POINT('',(1.52418692274867,-0.9,1.56359505313035));
#8543=CARTESIAN_POINT('',(1.66363611114492,0.5,3.15750657007714));
#8544=CARTESIAN_POINT('',(1.62877381404586,0.5,2.75902869084045));
#8545=CARTESIAN_POINT('',(1.66363611114492,-0.9,3.15750657007714));
#8546=CARTESIAN_POINT('Origin',(2.29124780561101,0.9,2.29954179168039));
#8547=CARTESIAN_POINT('',(1.3647777017174,0.9,3.18365329290144));
#8548=CARTESIAN_POINT('',(3.35716709790089,0.9,3.00934180740612));
#8549=CARTESIAN_POINT('',(3.35716709790089,0.9,3.00934180740612));
#8550=CARTESIAN_POINT('',(3.21771790950463,0.9,1.41543029045933));
#8551=CARTESIAN_POINT('',(3.21771790950463,0.9,1.41543029045933));
#8552=CARTESIAN_POINT('',(1.22532851332114,0.9,1.58974177595465));
#8553=CARTESIAN_POINT('',(1.22532851332114,0.9,1.58974177595465));
#8554=CARTESIAN_POINT('',(1.3647777017174,0.9,3.18365329290144));
#8555=CARTESIAN_POINT('Origin',(3.35716709790089,0.5,3.00934180740612));
#8556=CARTESIAN_POINT('',(3.21771790950463,0.5,1.41543029045933));
#8557=CARTESIAN_POINT('',(3.35716709790089,0.5,3.00934180740612));
#8558=CARTESIAN_POINT('',(3.21771790950463,0.5,1.41543029045933));
#8559=CARTESIAN_POINT('',(3.21771790950463,0.5,1.41543029045933));
#8560=CARTESIAN_POINT('',(3.35716709790089,0.5,3.00934180740612));
#8561=CARTESIAN_POINT('Origin',(2.29124780561101,0.5,2.29954179168039));
#8562=CARTESIAN_POINT('',(1.22532851332114,0.5,1.58974177595465));
#8563=CARTESIAN_POINT('',(3.35716709790089,0.5,3.00934180740612));
#8564=CARTESIAN_POINT('Origin',(0.747146023568809,-0.3,2.43463319293926));
#8565=CARTESIAN_POINT('',(1.26019081042021,-0.3,1.98821965519135));
#8566=CARTESIAN_POINT('',(1.32991540461833,-0.3,2.78517541366474));
#8567=CARTESIAN_POINT('',(1.26019081042021,-0.3,1.98821965519135));
#8568=CARTESIAN_POINT('',(0.480374109850668,-0.3,2.85950064615405));
#8569=CARTESIAN_POINT('',(0.0348622970990633,-0.3,2.8984778792367));
#8570=CARTESIAN_POINT('',(0.410649515652541,-0.3,2.06254488768065));
#8571=CARTESIAN_POINT('Origin',(0.,-0.3,2.5));
#8572=CARTESIAN_POINT('',(1.45942975003856,-0.3,1.97078850664181));
#8573=CARTESIAN_POINT('Origin',(0.0348622970990633,-0.3,2.8984778792367));
#8574=CARTESIAN_POINT('',(1.32991540461833,0.3,2.78517541366474));
#8575=CARTESIAN_POINT('',(1.32991540461833,-0.6,2.78517541366474));
#8576=CARTESIAN_POINT('',(0.480374109850668,0.3,2.85950064615405));
#8577=CARTESIAN_POINT('',(0.0348622970990633,0.3,2.8984778792367));
#8578=CARTESIAN_POINT('',(0.480374109850668,-0.48,2.85950064615405));
#8579=CARTESIAN_POINT('Origin',(0.747146023568809,0.3,2.43463319293926));
#8580=CARTESIAN_POINT('',(1.26019081042021,0.3,1.98821965519135));
#8581=CARTESIAN_POINT('',(1.26019081042021,0.3,1.98821965519135));
#8582=CARTESIAN_POINT('',(0.410649515652541,0.3,2.06254488768065));
#8583=CARTESIAN_POINT('',(1.45942975003856,0.3,1.97078850664181));
#8584=CARTESIAN_POINT('Origin',(0.,0.3,2.5));
#8585=CARTESIAN_POINT('Origin',(1.45942975003856,-0.3,1.97078850664181));
#8586=CARTESIAN_POINT('',(1.26019081042021,-0.6,1.98821965519135));
#8587=CARTESIAN_POINT('',(0.410649515652541,-0.48,2.06254488768065));
#8588=CARTESIAN_POINT('Origin',(0.,-0.48,2.5));
#8589=CARTESIAN_POINT('',(-0.6,0.48,2.5));
#8590=CARTESIAN_POINT('Origin',(0.,0.48,2.5));
#8591=CARTESIAN_POINT('',(-0.6,-0.48,2.5));
#8592=CARTESIAN_POINT('',(-0.6,-0.48,2.5));
#8593=CARTESIAN_POINT('Origin',(0.,-0.48,2.5));
#8594=CARTESIAN_POINT('Origin',(0.,0.48,2.5));
#8595=CARTESIAN_POINT('Origin',(0.,-0.48,2.5));
#8596=CARTESIAN_POINT('Origin',(3.21771790950463,-0.9,1.41543029045933));
#8597=CARTESIAN_POINT('',(3.21771790950463,-0.5,1.41543029045933));
#8598=CARTESIAN_POINT('',(1.22532851332114,-0.5,1.58974177595465));
#8599=CARTESIAN_POINT('',(3.21771790950463,-0.9,1.41543029045933));
#8600=CARTESIAN_POINT('',(3.21771790950463,-0.9,1.41543029045933));
#8601=CARTESIAN_POINT('',(1.22532851332114,-0.9,1.58974177595465));
#8602=CARTESIAN_POINT('',(1.22532851332114,-0.9,1.58974177595465));
#8603=CARTESIAN_POINT('',(1.22532851332114,-0.9,1.58974177595465));
#8604=CARTESIAN_POINT('Origin',(2.29124780561101,-0.5,2.29954179168039));
#8605=CARTESIAN_POINT('',(3.35716709790089,-0.5,3.00934180740612));
#8606=CARTESIAN_POINT('',(3.35716709790089,-0.5,3.00934180740612));
#8607=CARTESIAN_POINT('',(3.21771790950463,-0.5,1.41543029045933));
#8608=CARTESIAN_POINT('Origin',(1.22532851332114,-0.9,1.58974177595465));
#8609=CARTESIAN_POINT('',(1.3647777017174,-0.9,3.18365329290144));
#8610=CARTESIAN_POINT('',(1.3647777017174,-0.9,3.18365329290144));
#8611=CARTESIAN_POINT('',(1.3647777017174,-0.9,3.18365329290144));
#8612=CARTESIAN_POINT('Origin',(3.35716709790089,-0.9,3.00934180740612));
#8613=CARTESIAN_POINT('',(3.35716709790089,-0.9,3.00934180740612));
#8614=CARTESIAN_POINT('',(3.21771790950463,-0.9,1.41543029045933));
#8615=CARTESIAN_POINT('',(3.35716709790089,-0.9,3.00934180740612));
#8616=CARTESIAN_POINT('Origin',(1.3647777017174,-0.9,3.18365329290144));
#8617=CARTESIAN_POINT('',(3.35716709790089,-0.9,3.00934180740612));
#8618=CARTESIAN_POINT('Origin',(2.29124780561101,-0.9,2.29954179168039));
#9241=UNCERTAINTY_MEASURE_WITH_UNIT(LENGTH_MEASURE(0.001),#9286,
'DISTANCE_ACCURACY_VALUE',
'Maximum model space distance between geometric entities at asserted c
onnectivities');
#9255=UNCERTAINTY_MEASURE_WITH_UNIT(LENGTH_MEASURE(0.001),#9286,
'DISTANCE_ACCURACY_VALUE',
'Maximum model space distance between geometric entities at asserted c
onnectivities');
#9271=(
GEOMETRIC_REPRESENTATION_CONTEXT(3)
GLOBAL_UNCERTAINTY_ASSIGNED_CONTEXT((#9241))
GLOBAL_UNIT_ASSIGNED_CONTEXT((#9286,#9288,#9289))
REPRESENTATION_CONTEXT('','3D')
);
#9285=(
GEOMETRIC_REPRESENTATION_CONTEXT(3)
GLOBAL_UNCERTAINTY_ASSIGNED_CONTEXT((#9255))
GLOBAL_UNIT_ASSIGNED_CONTEXT((#9286,#9288,#9289))
REPRESENTATION_CONTEXT('','3D')
);
#9286=(
LENGTH_UNIT()
NAMED_UNIT(*)
SI_UNIT(.CENTI.,.METRE.)
);
#9288=(
NAMED_UNIT(*)
PLANE_ANGLE_UNIT()
SI_UNIT($,.RADIAN.)
);
#9289=(
NAMED_UNIT(*)
SI_UNIT($,.STERADIAN.)
SOLID_ANGLE_UNIT()
);
#9305=SHAPE_DEFINITION_REPRESENTATION(#9334,#9409);
#9334=PRODUCT_DEFINITION_SHAPE('',$,#9439);
#9409=SHAPE_REPRESENTATION('',(#5779),#9271);
#9423=PRODUCT_DEFINITION_CONTEXT('part definition',#9512,'design');
#9439=PRODUCT_DEFINITION('Operating lever','Operating lever',#9468,#9423);
#9468=PRODUCT_DEFINITION_FORMATION('',$,#9529);
#9512=APPLICATION_CONTEXT(
'Core Data for Automotive Mechanical Design Process');
#9513=PRODUCT_CONTEXT('part definition',#9512,'mechanical');
#9529=PRODUCT('Operating lever','Operating lever','Operating lever',(#9513));
#9592=COLOUR_RGB('Light Blue',0.38,0.62,0.78);
#9593=FILL_AREA_STYLE_COLOUR('',#9592);
#9594=FILL_AREA_STYLE('',(#9593));
#9595=SURFACE_STYLE_FILL_AREA(#9594);
#9596=SURFACE_SIDE_STYLE('',(#9595));
#9597=SURFACE_STYLE_USAGE(.BOTH.,#9596);
#9598=PRESENTATION_STYLE_ASSIGNMENT((#9597));
ENDSEC;
END-ISO-10303-21;
